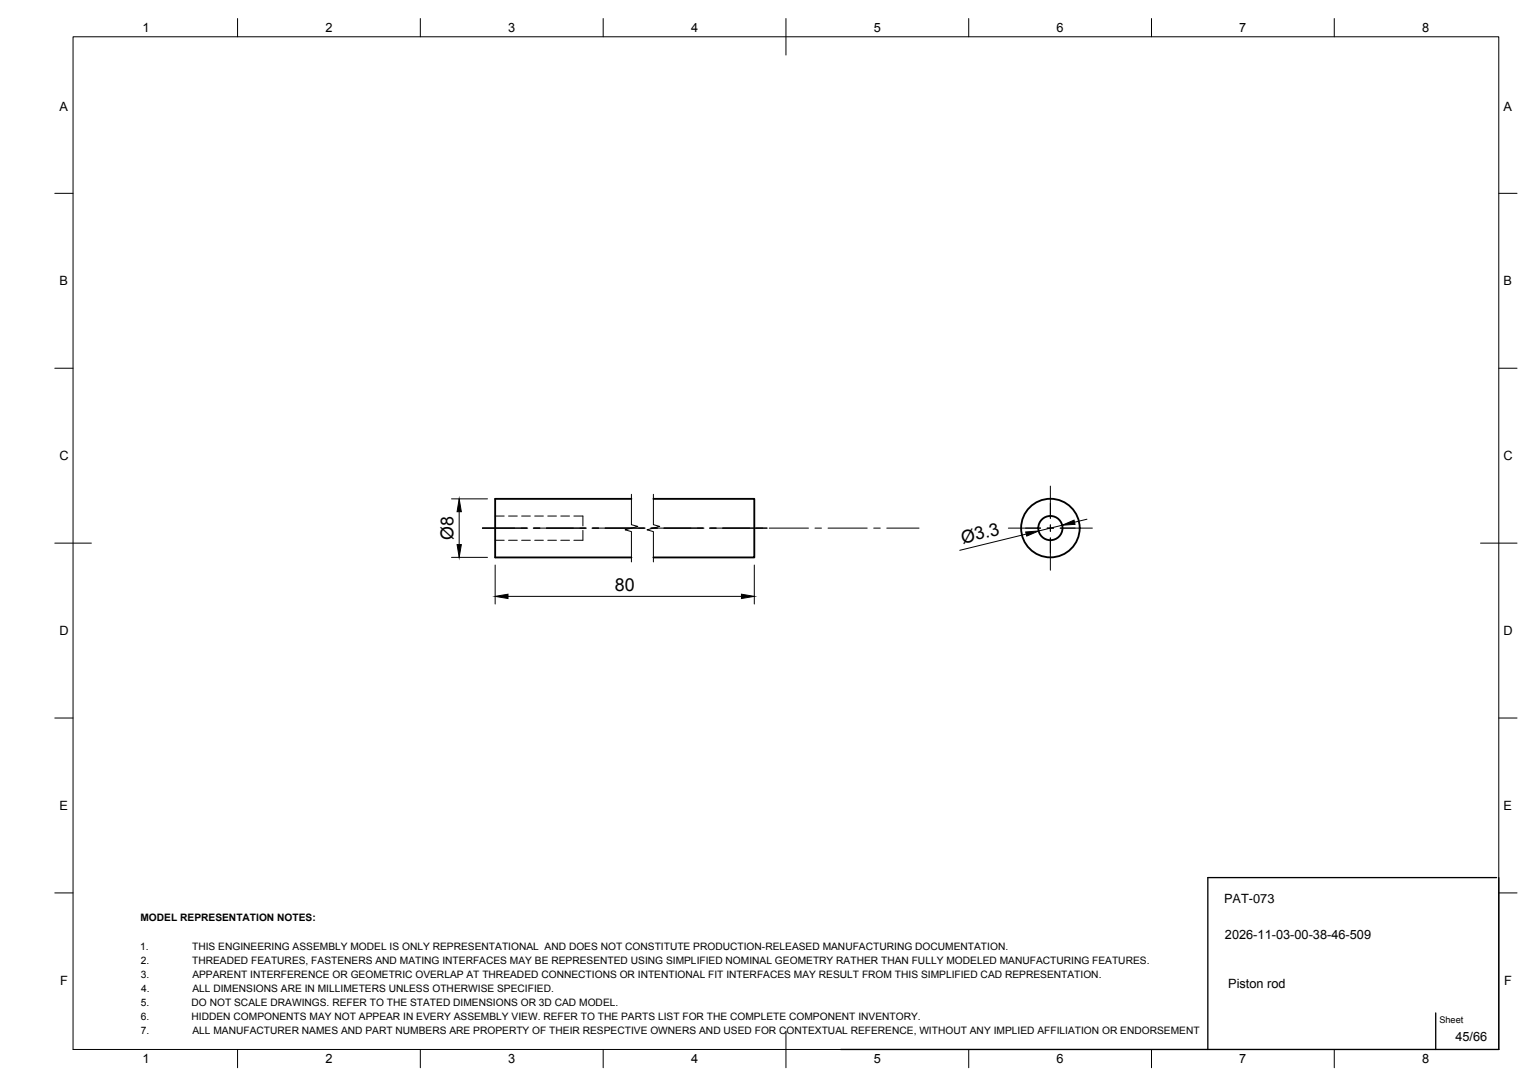
ISO-10303-21;
HEADER;
/* Generated by software containing ST-Developer
 * from STEP Tools, Inc. (www.steptools.com) 
 */

FILE_DESCRIPTION(
/* description */ ('Manual piston pump'),
/* implementation_level */ '2;1');

FILE_NAME(
/* name */ 'Piston rod.step',
/* time_stamp */ '2026-11-02T16:54:23-08:00',
/* author */ (''),
/* organization */ (''),
/* preprocessor_version */ 'ST-DEVELOPER v20.2',
/* originating_system */ 'Autodesk Translation Framework v15.17.0.0',
/* authorisation */ '');

FILE_SCHEMA (('AUTOMOTIVE_DESIGN { 1 0 10303 214 3 1 1 }'));
ENDSEC;

DATA;
#10=MECHANICAL_DESIGN_GEOMETRIC_PRESENTATION_REPRESENTATION('',(#736),#19043);
#602=SHAPE_REPRESENTATION_RELATIONSHIP('SRR','None',#19351,#665);
#665=ADVANCED_BREP_SHAPE_REPRESENTATION('',(#805),#19018);
#736=STYLED_ITEM('',(#19664),#805);
#805=MANIFOLD_SOLID_BREP('Body1',#9523);
#999=FACE_BOUND('',#2450,.T.);
#1236=CYLINDRICAL_SURFACE('',#11067,0.165);
#1237=CYLINDRICAL_SURFACE('',#11071,0.4);
#1699=FACE_OUTER_BOUND('',#2446,.T.);
#1700=FACE_OUTER_BOUND('',#2447,.T.);
#1701=FACE_OUTER_BOUND('',#2448,.T.);
#1702=FACE_OUTER_BOUND('',#2449,.T.);
#1703=FACE_OUTER_BOUND('',#2451,.T.);
#2446=EDGE_LOOP('',(#7931,#7932,#7933,#7934));
#2447=EDGE_LOOP('',(#7935));
#2448=EDGE_LOOP('',(#7936,#7937,#7938,#7939));
#2449=EDGE_LOOP('',(#7940));
#2450=EDGE_LOOP('',(#7941));
#2451=EDGE_LOOP('',(#7942));
#3022=CIRCLE('',#11068,0.165);
#3023=CIRCLE('',#11069,0.165);
#3024=CIRCLE('',#11072,0.4);
#3025=CIRCLE('',#11073,0.4);
#3571=LINE('',#17944,#4175);
#3572=LINE('',#17951,#4176);
#4175=VECTOR('',#13571,0.165);
#4176=VECTOR('',#13580,0.4);
#4913=VERTEX_POINT('',#17941);
#4914=VERTEX_POINT('',#17943);
#4915=VERTEX_POINT('',#17948);
#4916=VERTEX_POINT('',#17950);
#5952=EDGE_CURVE('',#4913,#4913,#3022,.T.);
#5953=EDGE_CURVE('',#4913,#4914,#3571,.T.);
#5954=EDGE_CURVE('',#4914,#4914,#3023,.T.);
#5955=EDGE_CURVE('',#4915,#4915,#3024,.T.);
#5956=EDGE_CURVE('',#4915,#4916,#3572,.T.);
#5957=EDGE_CURVE('',#4916,#4916,#3025,.T.);
#7931=ORIENTED_EDGE('',*,*,#5952,.F.);
#7932=ORIENTED_EDGE('',*,*,#5953,.T.);
#7933=ORIENTED_EDGE('',*,*,#5954,.F.);
#7934=ORIENTED_EDGE('',*,*,#5953,.F.);
#7935=ORIENTED_EDGE('',*,*,#5952,.T.);
#7936=ORIENTED_EDGE('',*,*,#5955,.F.);
#7937=ORIENTED_EDGE('',*,*,#5956,.T.);
#7938=ORIENTED_EDGE('',*,*,#5957,.T.);
#7939=ORIENTED_EDGE('',*,*,#5956,.F.);
#7940=ORIENTED_EDGE('',*,*,#5955,.T.);
#7941=ORIENTED_EDGE('',*,*,#5954,.T.);
#7942=ORIENTED_EDGE('',*,*,#5957,.F.);
#8795=PLANE('',#11070);
#8796=PLANE('',#11074);
#8797=PLANE('',#11075);
#9304=ADVANCED_FACE('',(#1699),#1236,.F.);
#9305=ADVANCED_FACE('',(#1700),#8795,.T.);
#9306=ADVANCED_FACE('',(#1701),#1237,.T.);
#9307=ADVANCED_FACE('',(#1702,#999),#8796,.T.);
#9308=ADVANCED_FACE('',(#1703),#8797,.F.);
#9523=CLOSED_SHELL('',(#9304,#9305,#9306,#9307,#9308));
#11066=AXIS2_PLACEMENT_3D('',#17939,#13565,#13566);
#11067=AXIS2_PLACEMENT_3D('',#17940,#13567,#13568);
#11068=AXIS2_PLACEMENT_3D('',#17942,#13569,#13570);
#11069=AXIS2_PLACEMENT_3D('',#17945,#13572,#13573);
#11070=AXIS2_PLACEMENT_3D('',#17946,#13574,#13575);
#11071=AXIS2_PLACEMENT_3D('',#17947,#13576,#13577);
#11072=AXIS2_PLACEMENT_3D('',#17949,#13578,#13579);
#11073=AXIS2_PLACEMENT_3D('',#17952,#13581,#13582);
#11074=AXIS2_PLACEMENT_3D('',#17953,#13583,#13584);
#11075=AXIS2_PLACEMENT_3D('',#17954,#13585,#13586);
#13565=DIRECTION('axis',(0.,0.,1.));
#13566=DIRECTION('refdir',(1.,0.,0.));
#13567=DIRECTION('center_axis',(0.,1.,0.));
#13568=DIRECTION('ref_axis',(1.,0.,0.));
#13569=DIRECTION('center_axis',(0.,1.,0.));
#13570=DIRECTION('ref_axis',(1.,0.,0.));
#13571=DIRECTION('',(0.,1.,0.));
#13572=DIRECTION('center_axis',(0.,-1.,0.));
#13573=DIRECTION('ref_axis',(1.,0.,0.));
#13574=DIRECTION('center_axis',(0.,1.,0.));
#13575=DIRECTION('ref_axis',(1.,0.,0.));
#13576=DIRECTION('center_axis',(0.,1.,0.));
#13577=DIRECTION('ref_axis',(1.,0.,0.));
#13578=DIRECTION('center_axis',(0.,1.,0.));
#13579=DIRECTION('ref_axis',(1.,0.,0.));
#13580=DIRECTION('',(0.,-1.,0.));
#13581=DIRECTION('center_axis',(0.,1.,0.));
#13582=DIRECTION('ref_axis',(1.,0.,0.));
#13583=DIRECTION('center_axis',(0.,1.,0.));
#13584=DIRECTION('ref_axis',(1.,0.,0.));
#13585=DIRECTION('center_axis',(0.,1.,0.));
#13586=DIRECTION('ref_axis',(1.,0.,0.));
#17939=CARTESIAN_POINT('',(0.,0.,0.));
#17940=CARTESIAN_POINT('Origin',(0.,1.2,4.5));
#17941=CARTESIAN_POINT('',(-0.165,1.2,4.5));
#17942=CARTESIAN_POINT('Origin',(0.,1.2,4.5));
#17943=CARTESIAN_POINT('',(-0.165,2.4,4.5));
#17944=CARTESIAN_POINT('',(-0.165,1.2,4.5));
#17945=CARTESIAN_POINT('Origin',(0.,2.4,4.5));
#17946=CARTESIAN_POINT('Origin',(0.,1.2,4.5));
#17947=CARTESIAN_POINT('Origin',(0.,-5.6,4.5));
#17948=CARTESIAN_POINT('',(-0.4,2.4,4.5));
#17949=CARTESIAN_POINT('Origin',(0.,2.4,4.5));
#17950=CARTESIAN_POINT('',(-0.4,-5.6,4.5));
#17951=CARTESIAN_POINT('',(-0.4,-5.6,4.5));
#17952=CARTESIAN_POINT('Origin',(0.,-5.6,4.5));
#17953=CARTESIAN_POINT('Origin',(0.,2.4,4.5));
#17954=CARTESIAN_POINT('Origin',(0.,-5.6,4.5));
#18947=UNCERTAINTY_MEASURE_WITH_UNIT(LENGTH_MEASURE(0.001),#19044,
'DISTANCE_ACCURACY_VALUE',
'Maximum model space distance between geometric entities at asserted c
onnectivities');
#18972=UNCERTAINTY_MEASURE_WITH_UNIT(LENGTH_MEASURE(0.001),#19044,
'DISTANCE_ACCURACY_VALUE',
'Maximum model space distance between geometric entities at asserted c
onnectivities');
#19018=(
GEOMETRIC_REPRESENTATION_CONTEXT(3)
GLOBAL_UNCERTAINTY_ASSIGNED_CONTEXT((#18947))
GLOBAL_UNIT_ASSIGNED_CONTEXT((#19044,#19046,#19047))
REPRESENTATION_CONTEXT('','3D')
);
#19043=(
GEOMETRIC_REPRESENTATION_CONTEXT(3)
GLOBAL_UNCERTAINTY_ASSIGNED_CONTEXT((#18972))
GLOBAL_UNIT_ASSIGNED_CONTEXT((#19044,#19046,#19047))
REPRESENTATION_CONTEXT('','3D')
);
#19044=(
LENGTH_UNIT()
NAMED_UNIT(*)
SI_UNIT(.CENTI.,.METRE.)
);
#19046=(
NAMED_UNIT(*)
PLANE_ANGLE_UNIT()
SI_UNIT($,.RADIAN.)
);
#19047=(
NAMED_UNIT(*)
SI_UNIT($,.STERADIAN.)
SOLID_ANGLE_UNIT()
);
#19093=SHAPE_DEFINITION_REPRESENTATION(#19170,#19351);
#19170=PRODUCT_DEFINITION_SHAPE('',$,#19422);
#19351=SHAPE_REPRESENTATION('',(#11066),#19018);
#19376=PRODUCT_DEFINITION_CONTEXT('part definition',#19588,'design');
#19422=PRODUCT_DEFINITION('2026-11-03-00-38-46-509','Piston rod',#19492,
#19376);
#19492=PRODUCT_DEFINITION_FORMATION('',$,#19635);
#19588=APPLICATION_CONTEXT(
'Core Data for Automotive Mechanical Design Process');
#19589=PRODUCT_CONTEXT('part definition',#19588,'mechanical');
#19635=PRODUCT('2026-11-03-00-38-46-509','Piston rod','Piston rod',(#19589));
#19664=PRESENTATION_STYLE_ASSIGNMENT((#19670));
#19670=SURFACE_STYLE_USAGE(.BOTH.,#19676);
#19676=SURFACE_SIDE_STYLE('',(#19682));
#19682=SURFACE_STYLE_FILL_AREA(#19688);
#19688=FILL_AREA_STYLE('CAD Library Painted - Steel gray',(#19694));
#19694=FILL_AREA_STYLE_COLOUR('CAD Library Painted - Steel gray',#19700);
#19700=COLOUR_RGB('CAD Library Painted - Steel gray',0.592156862745098,
0.631372549019608,0.67843137254902);
ENDSEC;
END-ISO-10303-21;
